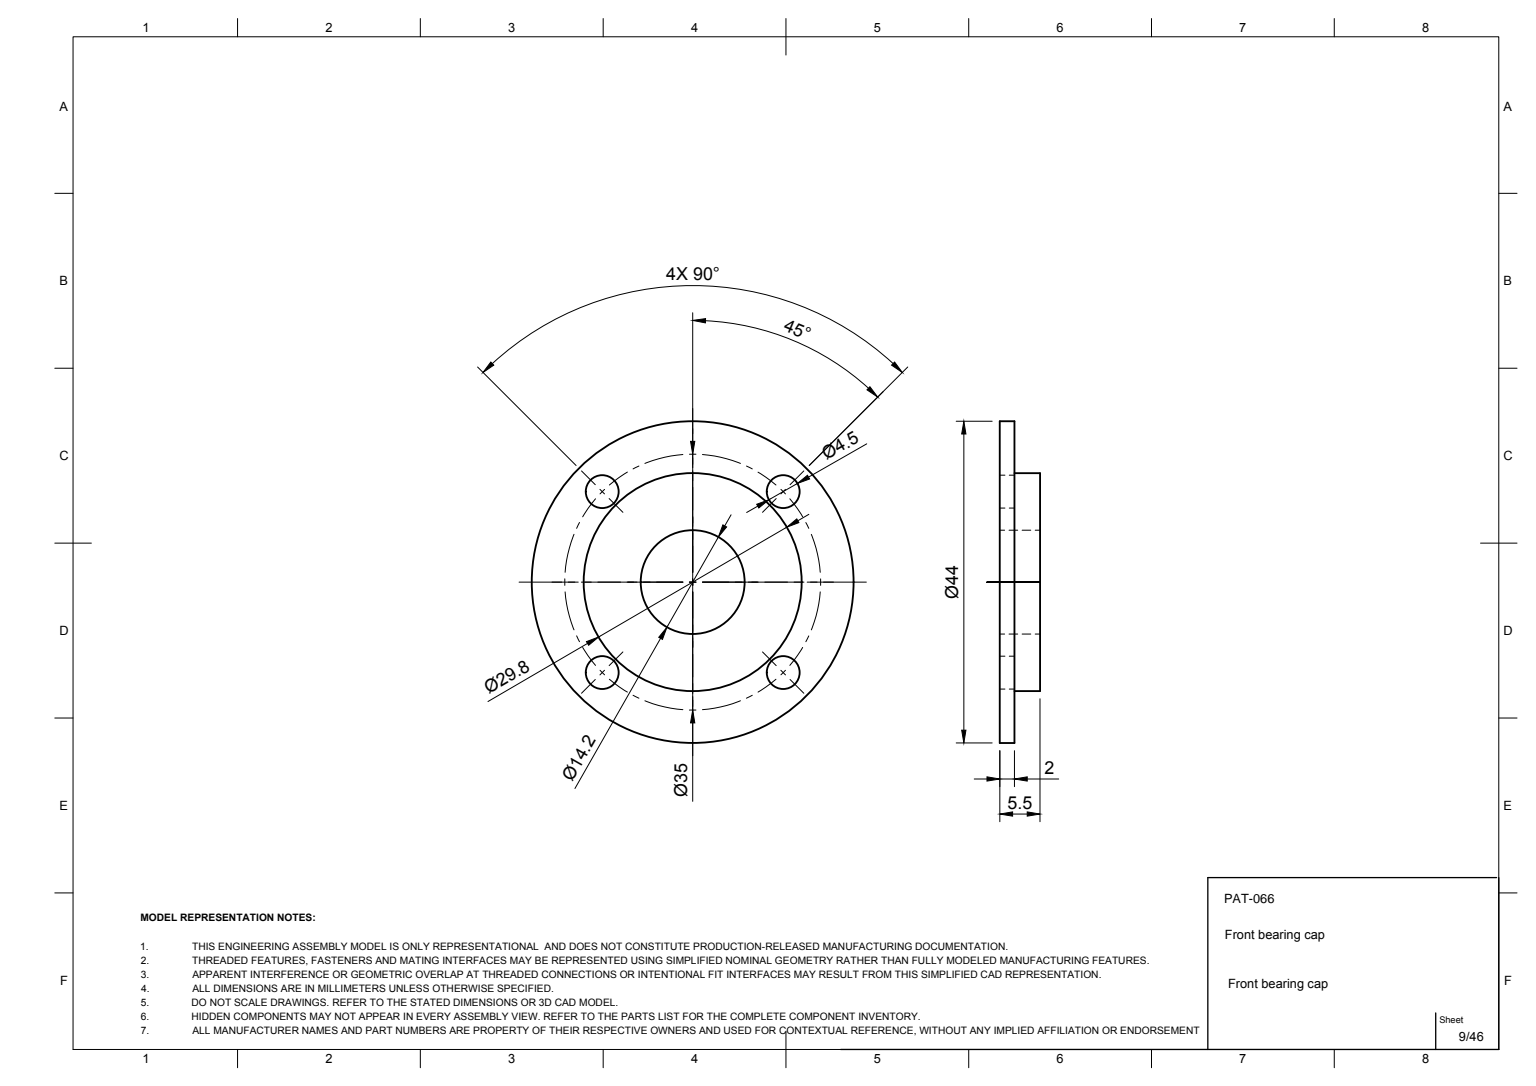
ISO-10303-21;
HEADER;
/* Generated by software containing ST-Developer
 * from STEP Tools, Inc. (www.steptools.com) 
 */

FILE_DESCRIPTION(
/* description */ ('Lever-operated bar clamp (toggle)'),
/* implementation_level */ '2;1');

FILE_NAME(
/* name */ 'Front bearing cap.step',
/* time_stamp */ '2026-10-28T03:25:02-07:00',
/* author */ (''),
/* organization */ (''),
/* preprocessor_version */ 'ST-DEVELOPER v20.2',
/* originating_system */ 'Autodesk Translation Framework v15.17.0.0',
/* authorisation */ '');

FILE_SCHEMA (('AUTOMOTIVE_DESIGN { 1 0 10303 214 3 1 1 }'));
ENDSEC;

DATA;
#10=MECHANICAL_DESIGN_GEOMETRIC_PRESENTATION_REPRESENTATION('',(#414),#12413);
#338=SHAPE_REPRESENTATION_RELATIONSHIP('SRR','None',#12577,#376);
#376=ADVANCED_BREP_SHAPE_REPRESENTATION('',(#461),#12374);
#414=STYLED_ITEM('',(#12869),#461);
#461=MANIFOLD_SOLID_BREP('Body1',#6573);
#544=FACE_BOUND('',#1408,.T.);
#545=FACE_BOUND('',#1412,.T.);
#546=FACE_BOUND('',#1413,.T.);
#547=FACE_BOUND('',#1414,.T.);
#548=FACE_BOUND('',#1415,.T.);
#549=FACE_BOUND('',#1416,.T.);
#550=FACE_BOUND('',#1418,.T.);
#551=FACE_BOUND('',#1419,.T.);
#552=FACE_BOUND('',#1420,.T.);
#553=FACE_BOUND('',#1421,.T.);
#554=FACE_BOUND('',#1422,.T.);
#689=PLANE('',#7177);
#690=PLANE('',#7184);
#691=PLANE('',#7185);
#952=FACE_OUTER_BOUND('',#1402,.T.);
#953=FACE_OUTER_BOUND('',#1403,.T.);
#954=FACE_OUTER_BOUND('',#1404,.T.);
#955=FACE_OUTER_BOUND('',#1405,.T.);
#956=FACE_OUTER_BOUND('',#1406,.T.);
#957=FACE_OUTER_BOUND('',#1407,.T.);
#958=FACE_OUTER_BOUND('',#1409,.T.);
#959=FACE_OUTER_BOUND('',#1410,.T.);
#960=FACE_OUTER_BOUND('',#1411,.T.);
#961=FACE_OUTER_BOUND('',#1417,.T.);
#1402=EDGE_LOOP('',(#4721,#4722,#4723,#4724));
#1403=EDGE_LOOP('',(#4725,#4726,#4727,#4728));
#1404=EDGE_LOOP('',(#4729,#4730,#4731,#4732));
#1405=EDGE_LOOP('',(#4733,#4734,#4735,#4736));
#1406=EDGE_LOOP('',(#4737,#4738,#4739,#4740));
#1407=EDGE_LOOP('',(#4741));
#1408=EDGE_LOOP('',(#4742));
#1409=EDGE_LOOP('',(#4743,#4744,#4745,#4746));
#1410=EDGE_LOOP('',(#4747,#4748,#4749,#4750));
#1411=EDGE_LOOP('',(#4751));
#1412=EDGE_LOOP('',(#4752));
#1413=EDGE_LOOP('',(#4753));
#1414=EDGE_LOOP('',(#4754));
#1415=EDGE_LOOP('',(#4755));
#1416=EDGE_LOOP('',(#4756));
#1417=EDGE_LOOP('',(#4757));
#1418=EDGE_LOOP('',(#4758));
#1419=EDGE_LOOP('',(#4759));
#1420=EDGE_LOOP('',(#4760));
#1421=EDGE_LOOP('',(#4761));
#1422=EDGE_LOOP('',(#4762));
#1949=LINE('',#10370,#2390);
#1950=LINE('',#10376,#2391);
#1951=LINE('',#10382,#2392);
#1952=LINE('',#10388,#2393);
#1953=LINE('',#10394,#2394);
#1954=LINE('',#10401,#2395);
#1955=LINE('',#10407,#2396);
#2390=VECTOR('',#8242,0.225);
#2391=VECTOR('',#8249,0.225);
#2392=VECTOR('',#8256,0.225);
#2393=VECTOR('',#8263,0.225);
#2394=VECTOR('',#8270,1.49);
#2395=VECTOR('',#8279,0.71);
#2396=VECTOR('',#8286,2.2);
#2785=CIRCLE('',#7163,0.225);
#2786=CIRCLE('',#7164,0.225);
#2787=CIRCLE('',#7166,0.225);
#2788=CIRCLE('',#7167,0.225);
#2789=CIRCLE('',#7169,0.225);
#2790=CIRCLE('',#7170,0.225);
#2791=CIRCLE('',#7172,0.225);
#2792=CIRCLE('',#7173,0.225);
#2793=CIRCLE('',#7175,1.49);
#2794=CIRCLE('',#7176,1.49);
#2795=CIRCLE('',#7178,0.71);
#2796=CIRCLE('',#7180,0.71);
#2797=CIRCLE('',#7182,2.2);
#2798=CIRCLE('',#7183,2.2);
#3174=VERTEX_POINT('',#10367);
#3175=VERTEX_POINT('',#10369);
#3176=VERTEX_POINT('',#10373);
#3177=VERTEX_POINT('',#10375);
#3178=VERTEX_POINT('',#10379);
#3179=VERTEX_POINT('',#10381);
#3180=VERTEX_POINT('',#10385);
#3181=VERTEX_POINT('',#10387);
#3182=VERTEX_POINT('',#10391);
#3183=VERTEX_POINT('',#10393);
#3184=VERTEX_POINT('',#10397);
#3185=VERTEX_POINT('',#10400);
#3186=VERTEX_POINT('',#10404);
#3187=VERTEX_POINT('',#10406);
#3765=EDGE_CURVE('',#3174,#3174,#2785,.T.);
#3766=EDGE_CURVE('',#3174,#3175,#1949,.T.);
#3767=EDGE_CURVE('',#3175,#3175,#2786,.T.);
#3768=EDGE_CURVE('',#3176,#3176,#2787,.T.);
#3769=EDGE_CURVE('',#3176,#3177,#1950,.T.);
#3770=EDGE_CURVE('',#3177,#3177,#2788,.T.);
#3771=EDGE_CURVE('',#3178,#3178,#2789,.T.);
#3772=EDGE_CURVE('',#3178,#3179,#1951,.T.);
#3773=EDGE_CURVE('',#3179,#3179,#2790,.T.);
#3774=EDGE_CURVE('',#3180,#3180,#2791,.T.);
#3775=EDGE_CURVE('',#3180,#3181,#1952,.T.);
#3776=EDGE_CURVE('',#3181,#3181,#2792,.T.);
#3777=EDGE_CURVE('',#3182,#3182,#2793,.T.);
#3778=EDGE_CURVE('',#3182,#3183,#1953,.T.);
#3779=EDGE_CURVE('',#3183,#3183,#2794,.T.);
#3780=EDGE_CURVE('',#3184,#3184,#2795,.T.);
#3781=EDGE_CURVE('',#3184,#3185,#1954,.T.);
#3782=EDGE_CURVE('',#3185,#3185,#2796,.T.);
#3783=EDGE_CURVE('',#3186,#3186,#2797,.T.);
#3784=EDGE_CURVE('',#3186,#3187,#1955,.T.);
#3785=EDGE_CURVE('',#3187,#3187,#2798,.T.);
#4721=ORIENTED_EDGE('',*,*,#3765,.F.);
#4722=ORIENTED_EDGE('',*,*,#3766,.T.);
#4723=ORIENTED_EDGE('',*,*,#3767,.F.);
#4724=ORIENTED_EDGE('',*,*,#3766,.F.);
#4725=ORIENTED_EDGE('',*,*,#3768,.F.);
#4726=ORIENTED_EDGE('',*,*,#3769,.T.);
#4727=ORIENTED_EDGE('',*,*,#3770,.F.);
#4728=ORIENTED_EDGE('',*,*,#3769,.F.);
#4729=ORIENTED_EDGE('',*,*,#3771,.F.);
#4730=ORIENTED_EDGE('',*,*,#3772,.T.);
#4731=ORIENTED_EDGE('',*,*,#3773,.F.);
#4732=ORIENTED_EDGE('',*,*,#3772,.F.);
#4733=ORIENTED_EDGE('',*,*,#3774,.F.);
#4734=ORIENTED_EDGE('',*,*,#3775,.T.);
#4735=ORIENTED_EDGE('',*,*,#3776,.F.);
#4736=ORIENTED_EDGE('',*,*,#3775,.F.);
#4737=ORIENTED_EDGE('',*,*,#3777,.F.);
#4738=ORIENTED_EDGE('',*,*,#3778,.T.);
#4739=ORIENTED_EDGE('',*,*,#3779,.F.);
#4740=ORIENTED_EDGE('',*,*,#3778,.F.);
#4741=ORIENTED_EDGE('',*,*,#3777,.T.);
#4742=ORIENTED_EDGE('',*,*,#3780,.T.);
#4743=ORIENTED_EDGE('',*,*,#3780,.F.);
#4744=ORIENTED_EDGE('',*,*,#3781,.T.);
#4745=ORIENTED_EDGE('',*,*,#3782,.T.);
#4746=ORIENTED_EDGE('',*,*,#3781,.F.);
#4747=ORIENTED_EDGE('',*,*,#3783,.F.);
#4748=ORIENTED_EDGE('',*,*,#3784,.T.);
#4749=ORIENTED_EDGE('',*,*,#3785,.T.);
#4750=ORIENTED_EDGE('',*,*,#3784,.F.);
#4751=ORIENTED_EDGE('',*,*,#3783,.T.);
#4752=ORIENTED_EDGE('',*,*,#3779,.T.);
#4753=ORIENTED_EDGE('',*,*,#3776,.T.);
#4754=ORIENTED_EDGE('',*,*,#3773,.T.);
#4755=ORIENTED_EDGE('',*,*,#3770,.T.);
#4756=ORIENTED_EDGE('',*,*,#3767,.T.);
#4757=ORIENTED_EDGE('',*,*,#3785,.F.);
#4758=ORIENTED_EDGE('',*,*,#3782,.F.);
#4759=ORIENTED_EDGE('',*,*,#3774,.T.);
#4760=ORIENTED_EDGE('',*,*,#3771,.T.);
#4761=ORIENTED_EDGE('',*,*,#3768,.T.);
#4762=ORIENTED_EDGE('',*,*,#3765,.T.);
#6059=CYLINDRICAL_SURFACE('',#7162,0.225);
#6060=CYLINDRICAL_SURFACE('',#7165,0.225);
#6061=CYLINDRICAL_SURFACE('',#7168,0.225);
#6062=CYLINDRICAL_SURFACE('',#7171,0.225);
#6063=CYLINDRICAL_SURFACE('',#7174,1.49);
#6064=CYLINDRICAL_SURFACE('',#7179,0.71);
#6065=CYLINDRICAL_SURFACE('',#7181,2.2);
#6227=ADVANCED_FACE('',(#952),#6059,.F.);
#6228=ADVANCED_FACE('',(#953),#6060,.F.);
#6229=ADVANCED_FACE('',(#954),#6061,.F.);
#6230=ADVANCED_FACE('',(#955),#6062,.F.);
#6231=ADVANCED_FACE('',(#956),#6063,.T.);
#6232=ADVANCED_FACE('',(#957,#544),#689,.T.);
#6233=ADVANCED_FACE('',(#958),#6064,.F.);
#6234=ADVANCED_FACE('',(#959),#6065,.T.);
#6235=ADVANCED_FACE('',(#960,#545,#546,#547,#548,#549),#690,.T.);
#6236=ADVANCED_FACE('',(#961,#550,#551,#552,#553,#554),#691,.F.);
#6573=CLOSED_SHELL('',(#6227,#6228,#6229,#6230,#6231,#6232,#6233,#6234,
#6235,#6236));
#7161=AXIS2_PLACEMENT_3D('',#10365,#8236,#8237);
#7162=AXIS2_PLACEMENT_3D('',#10366,#8238,#8239);
#7163=AXIS2_PLACEMENT_3D('',#10368,#8240,#8241);
#7164=AXIS2_PLACEMENT_3D('',#10371,#8243,#8244);
#7165=AXIS2_PLACEMENT_3D('',#10372,#8245,#8246);
#7166=AXIS2_PLACEMENT_3D('',#10374,#8247,#8248);
#7167=AXIS2_PLACEMENT_3D('',#10377,#8250,#8251);
#7168=AXIS2_PLACEMENT_3D('',#10378,#8252,#8253);
#7169=AXIS2_PLACEMENT_3D('',#10380,#8254,#8255);
#7170=AXIS2_PLACEMENT_3D('',#10383,#8257,#8258);
#7171=AXIS2_PLACEMENT_3D('',#10384,#8259,#8260);
#7172=AXIS2_PLACEMENT_3D('',#10386,#8261,#8262);
#7173=AXIS2_PLACEMENT_3D('',#10389,#8264,#8265);
#7174=AXIS2_PLACEMENT_3D('',#10390,#8266,#8267);
#7175=AXIS2_PLACEMENT_3D('',#10392,#8268,#8269);
#7176=AXIS2_PLACEMENT_3D('',#10395,#8271,#8272);
#7177=AXIS2_PLACEMENT_3D('',#10396,#8273,#8274);
#7178=AXIS2_PLACEMENT_3D('',#10398,#8275,#8276);
#7179=AXIS2_PLACEMENT_3D('',#10399,#8277,#8278);
#7180=AXIS2_PLACEMENT_3D('',#10402,#8280,#8281);
#7181=AXIS2_PLACEMENT_3D('',#10403,#8282,#8283);
#7182=AXIS2_PLACEMENT_3D('',#10405,#8284,#8285);
#7183=AXIS2_PLACEMENT_3D('',#10408,#8287,#8288);
#7184=AXIS2_PLACEMENT_3D('',#10409,#8289,#8290);
#7185=AXIS2_PLACEMENT_3D('',#10410,#8291,#8292);
#8236=DIRECTION('axis',(0.,0.,1.));
#8237=DIRECTION('refdir',(1.,0.,0.));
#8238=DIRECTION('center_axis',(0.,1.,0.));
#8239=DIRECTION('ref_axis',(1.,0.,0.));
#8240=DIRECTION('center_axis',(0.,1.,0.));
#8241=DIRECTION('ref_axis',(1.,0.,0.));
#8242=DIRECTION('',(0.,1.,0.));
#8243=DIRECTION('center_axis',(0.,-1.,0.));
#8244=DIRECTION('ref_axis',(1.,0.,0.));
#8245=DIRECTION('center_axis',(0.,1.,0.));
#8246=DIRECTION('ref_axis',(1.,0.,0.));
#8247=DIRECTION('center_axis',(0.,1.,0.));
#8248=DIRECTION('ref_axis',(1.,0.,0.));
#8249=DIRECTION('',(0.,1.,0.));
#8250=DIRECTION('center_axis',(0.,-1.,0.));
#8251=DIRECTION('ref_axis',(1.,0.,0.));
#8252=DIRECTION('center_axis',(0.,1.,0.));
#8253=DIRECTION('ref_axis',(1.,0.,0.));
#8254=DIRECTION('center_axis',(0.,1.,0.));
#8255=DIRECTION('ref_axis',(1.,0.,0.));
#8256=DIRECTION('',(0.,1.,0.));
#8257=DIRECTION('center_axis',(0.,-1.,0.));
#8258=DIRECTION('ref_axis',(1.,0.,0.));
#8259=DIRECTION('center_axis',(0.,1.,0.));
#8260=DIRECTION('ref_axis',(1.,0.,0.));
#8261=DIRECTION('center_axis',(0.,1.,0.));
#8262=DIRECTION('ref_axis',(1.,0.,0.));
#8263=DIRECTION('',(0.,1.,0.));
#8264=DIRECTION('center_axis',(0.,-1.,0.));
#8265=DIRECTION('ref_axis',(1.,0.,0.));
#8266=DIRECTION('center_axis',(0.,1.,0.));
#8267=DIRECTION('ref_axis',(1.,0.,0.));
#8268=DIRECTION('center_axis',(0.,1.,0.));
#8269=DIRECTION('ref_axis',(1.,0.,0.));
#8270=DIRECTION('',(0.,-1.,0.));
#8271=DIRECTION('center_axis',(0.,-1.,0.));
#8272=DIRECTION('ref_axis',(1.,0.,0.));
#8273=DIRECTION('center_axis',(0.,1.,0.));
#8274=DIRECTION('ref_axis',(1.,0.,0.));
#8275=DIRECTION('center_axis',(0.,-1.,0.));
#8276=DIRECTION('ref_axis',(1.,0.,0.));
#8277=DIRECTION('center_axis',(0.,1.,0.));
#8278=DIRECTION('ref_axis',(1.,0.,0.));
#8279=DIRECTION('',(0.,-1.,0.));
#8280=DIRECTION('center_axis',(0.,-1.,0.));
#8281=DIRECTION('ref_axis',(1.,0.,0.));
#8282=DIRECTION('center_axis',(0.,1.,0.));
#8283=DIRECTION('ref_axis',(1.,0.,0.));
#8284=DIRECTION('center_axis',(0.,1.,0.));
#8285=DIRECTION('ref_axis',(1.,0.,0.));
#8286=DIRECTION('',(0.,-1.,0.));
#8287=DIRECTION('center_axis',(0.,1.,0.));
#8288=DIRECTION('ref_axis',(1.,0.,0.));
#8289=DIRECTION('center_axis',(0.,1.,0.));
#8290=DIRECTION('ref_axis',(1.,0.,0.));
#8291=DIRECTION('center_axis',(0.,1.,0.));
#8292=DIRECTION('ref_axis',(1.,0.,0.));
#10365=CARTESIAN_POINT('',(0.,0.,0.));
#10366=CARTESIAN_POINT('Origin',(-5.23743686707646,-1.1,9.76256313292354));
#10367=CARTESIAN_POINT('',(-5.46243686707646,-1.,9.76256313292354));
#10368=CARTESIAN_POINT('Origin',(-5.23743686707646,-1.,9.76256313292354));
#10369=CARTESIAN_POINT('',(-5.46243686707646,-0.8,9.76256313292354));
#10370=CARTESIAN_POINT('',(-5.46243686707646,-1.1,9.76256313292354));
#10371=CARTESIAN_POINT('Origin',(-5.23743686707646,-0.8,9.76256313292354));
#10372=CARTESIAN_POINT('Origin',(-5.23743686707646,-1.1,12.2374368670765));
#10373=CARTESIAN_POINT('',(-5.46243686707646,-1.,12.2374368670765));
#10374=CARTESIAN_POINT('Origin',(-5.23743686707646,-1.,12.2374368670765));
#10375=CARTESIAN_POINT('',(-5.46243686707646,-0.8,12.2374368670765));
#10376=CARTESIAN_POINT('',(-5.46243686707646,-1.1,12.2374368670765));
#10377=CARTESIAN_POINT('Origin',(-5.23743686707646,-0.8,12.2374368670765));
#10378=CARTESIAN_POINT('Origin',(-2.76256313292354,-1.1,12.2374368670765));
#10379=CARTESIAN_POINT('',(-2.98756313292354,-1.,12.2374368670765));
#10380=CARTESIAN_POINT('Origin',(-2.76256313292354,-1.,12.2374368670765));
#10381=CARTESIAN_POINT('',(-2.98756313292354,-0.8,12.2374368670765));
#10382=CARTESIAN_POINT('',(-2.98756313292354,-1.1,12.2374368670765));
#10383=CARTESIAN_POINT('Origin',(-2.76256313292354,-0.8,12.2374368670765));
#10384=CARTESIAN_POINT('Origin',(-2.76256313292354,-1.1,9.76256313292354));
#10385=CARTESIAN_POINT('',(-2.98756313292354,-1.,9.76256313292354));
#10386=CARTESIAN_POINT('Origin',(-2.76256313292354,-1.,9.76256313292354));
#10387=CARTESIAN_POINT('',(-2.98756313292354,-0.8,9.76256313292354));
#10388=CARTESIAN_POINT('',(-2.98756313292354,-1.1,9.76256313292354));
#10389=CARTESIAN_POINT('Origin',(-2.76256313292354,-0.8,9.76256313292354));
#10390=CARTESIAN_POINT('Origin',(-4.,-0.8,11.));
#10391=CARTESIAN_POINT('',(-5.49,-0.45,11.));
#10392=CARTESIAN_POINT('Origin',(-4.,-0.45,11.));
#10393=CARTESIAN_POINT('',(-5.49,-0.8,11.));
#10394=CARTESIAN_POINT('',(-5.49,-0.8,11.));
#10395=CARTESIAN_POINT('Origin',(-4.,-0.8,11.));
#10396=CARTESIAN_POINT('Origin',(-4.,-0.45,11.));
#10397=CARTESIAN_POINT('',(-4.71,-0.45,11.));
#10398=CARTESIAN_POINT('Origin',(-4.,-0.45,11.));
#10399=CARTESIAN_POINT('Origin',(-4.,-1.,11.));
#10400=CARTESIAN_POINT('',(-4.71,-1.,11.));
#10401=CARTESIAN_POINT('',(-4.71,-1.,11.));
#10402=CARTESIAN_POINT('Origin',(-4.,-1.,11.));
#10403=CARTESIAN_POINT('Origin',(-4.,-1.,11.));
#10404=CARTESIAN_POINT('',(-6.2,-0.8,11.));
#10405=CARTESIAN_POINT('Origin',(-4.,-0.8,11.));
#10406=CARTESIAN_POINT('',(-6.2,-1.,11.));
#10407=CARTESIAN_POINT('',(-6.2,-1.,11.));
#10408=CARTESIAN_POINT('Origin',(-4.,-1.,11.));
#10409=CARTESIAN_POINT('Origin',(-4.,-0.8,11.));
#10410=CARTESIAN_POINT('Origin',(-4.,-1.,11.));
#12328=UNCERTAINTY_MEASURE_WITH_UNIT(LENGTH_MEASURE(0.001),#12414,
'DISTANCE_ACCURACY_VALUE',
'Maximum model space distance between geometric entities at asserted c
onnectivities');
#12367=UNCERTAINTY_MEASURE_WITH_UNIT(LENGTH_MEASURE(0.001),#12414,
'DISTANCE_ACCURACY_VALUE',
'Maximum model space distance between geometric entities at asserted c
onnectivities');
#12374=(
GEOMETRIC_REPRESENTATION_CONTEXT(3)
GLOBAL_UNCERTAINTY_ASSIGNED_CONTEXT((#12328))
GLOBAL_UNIT_ASSIGNED_CONTEXT((#12414,#12416,#12417))
REPRESENTATION_CONTEXT('','3D')
);
#12413=(
GEOMETRIC_REPRESENTATION_CONTEXT(3)
GLOBAL_UNCERTAINTY_ASSIGNED_CONTEXT((#12367))
GLOBAL_UNIT_ASSIGNED_CONTEXT((#12414,#12416,#12417))
REPRESENTATION_CONTEXT('','3D')
);
#12414=(
LENGTH_UNIT()
NAMED_UNIT(*)
SI_UNIT(.CENTI.,.METRE.)
);
#12416=(
NAMED_UNIT(*)
PLANE_ANGLE_UNIT()
SI_UNIT($,.RADIAN.)
);
#12417=(
NAMED_UNIT(*)
SI_UNIT($,.STERADIAN.)
SOLID_ANGLE_UNIT()
);
#12424=SHAPE_DEFINITION_REPRESENTATION(#12469,#12577);
#12469=PRODUCT_DEFINITION_SHAPE('',$,#12623);
#12577=SHAPE_REPRESENTATION('',(#7161),#12374);
#12616=PRODUCT_DEFINITION_CONTEXT('part definition',#12753,'design');
#12623=PRODUCT_DEFINITION('Front bearing cap','Front bearing cap',#12668,
#12616);
#12668=PRODUCT_DEFINITION_FORMATION('',$,#12761);
#12753=APPLICATION_CONTEXT(
'Core Data for Automotive Mechanical Design Process');
#12754=PRODUCT_CONTEXT('part definition',#12753,'mechanical');
#12761=PRODUCT('Front bearing cap','Front bearing cap',
'Front bearing cap',(#12754));
#12863=COLOUR_RGB('Grey',0.48,0.52,0.57);
#12864=FILL_AREA_STYLE_COLOUR('',#12863);
#12865=FILL_AREA_STYLE('',(#12864));
#12866=SURFACE_STYLE_FILL_AREA(#12865);
#12867=SURFACE_SIDE_STYLE('',(#12866));
#12868=SURFACE_STYLE_USAGE(.BOTH.,#12867);
#12869=PRESENTATION_STYLE_ASSIGNMENT((#12868));
ENDSEC;
END-ISO-10303-21;
